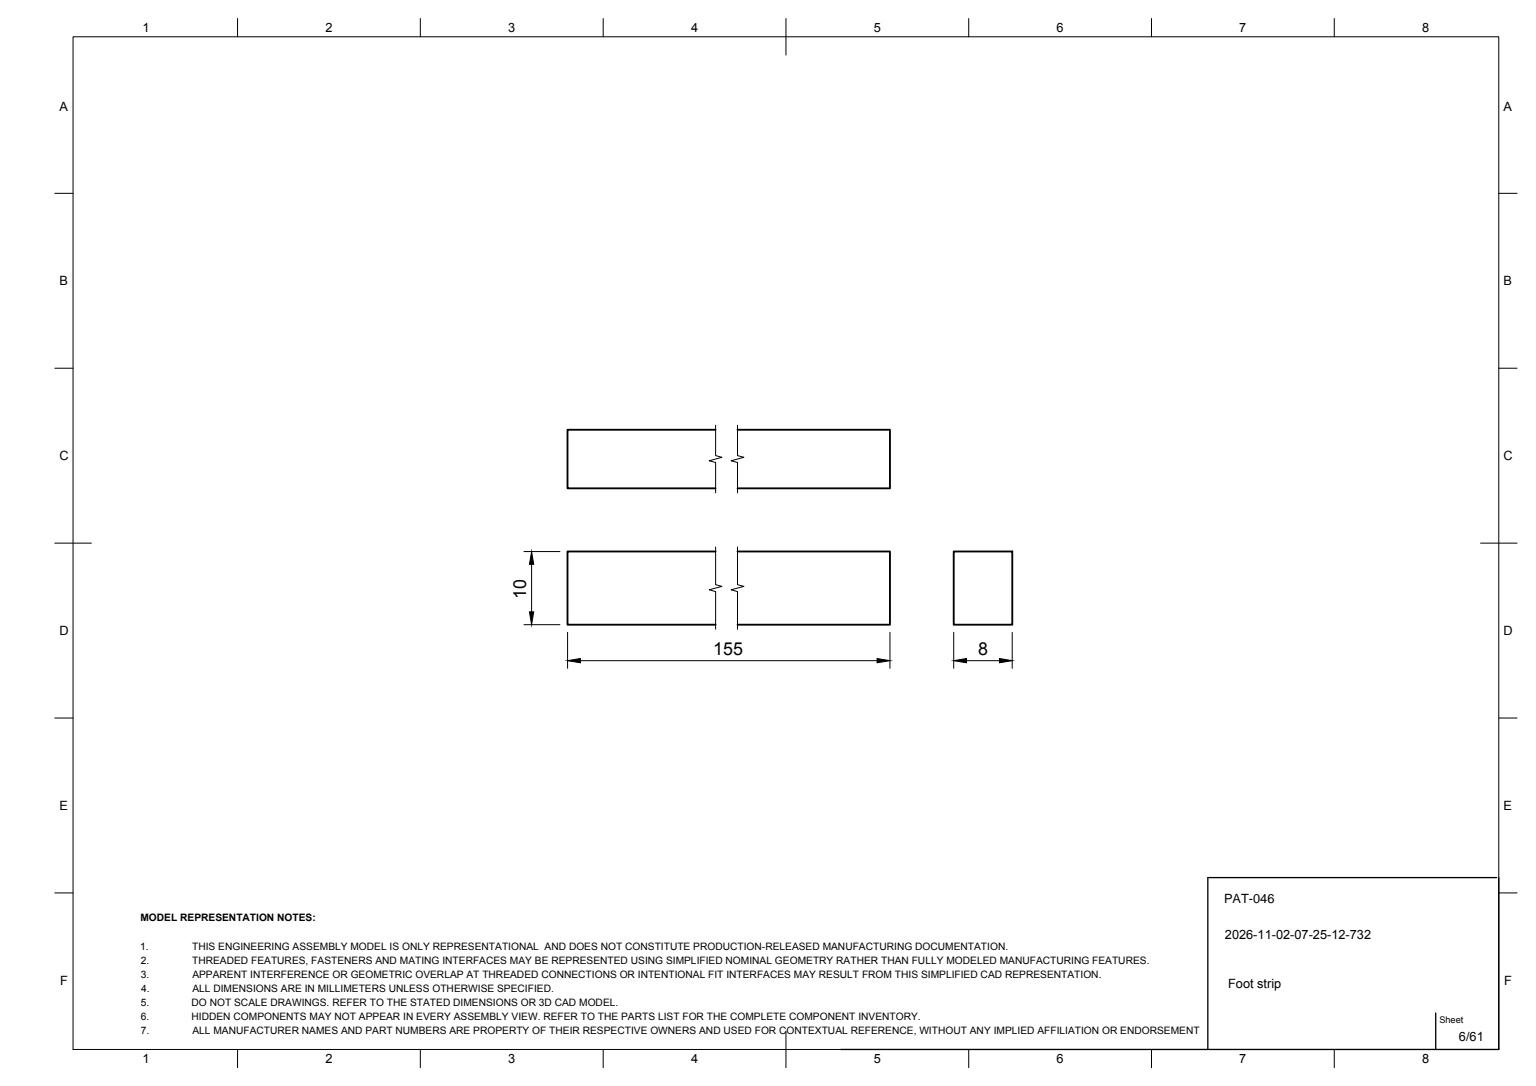
ISO-10303-21;
HEADER;
/* Generated by software containing ST-Developer
 * from STEP Tools, Inc. (www.steptools.com) 
 */

FILE_DESCRIPTION(
/* description */ ('Gear mesh backlash fixture'),
/* implementation_level */ '2;1');

FILE_NAME(
/* name */ 'Foot strip.step',
/* time_stamp */ '2026-10-28T03:26:00-07:00',
/* author */ (''),
/* organization */ (''),
/* preprocessor_version */ 'ST-DEVELOPER v20.2',
/* originating_system */ 'Autodesk Translation Framework v15.17.0.0',
/* authorisation */ '');

FILE_SCHEMA (('AUTOMOTIVE_DESIGN { 1 0 10303 214 3 1 1 }'));
ENDSEC;

DATA;
#10=MECHANICAL_DESIGN_GEOMETRIC_PRESENTATION_REPRESENTATION('',(#1017),#57900);
#917=SHAPE_REPRESENTATION_RELATIONSHIP('SRR','None',#58112,#967);
#967=ADVANCED_BREP_SHAPE_REPRESENTATION('',(#1082),#57845);
#1017=STYLED_ITEM('',(#58451),#1082);
#1082=MANIFOLD_SOLID_BREP('Body1',#13577);
#1336=PLANE('',#14241);
#1337=PLANE('',#14242);
#1338=PLANE('',#14243);
#1339=PLANE('',#14244);
#1340=PLANE('',#14245);
#1341=PLANE('',#14246);
#1712=FACE_OUTER_BOUND('',#2501,.T.);
#1713=FACE_OUTER_BOUND('',#2502,.T.);
#1714=FACE_OUTER_BOUND('',#2503,.T.);
#1715=FACE_OUTER_BOUND('',#2504,.T.);
#1716=FACE_OUTER_BOUND('',#2505,.T.);
#1717=FACE_OUTER_BOUND('',#2506,.T.);
#2501=EDGE_LOOP('',(#8975,#8976,#8977,#8978));
#2502=EDGE_LOOP('',(#8979,#8980,#8981,#8982));
#2503=EDGE_LOOP('',(#8983,#8984,#8985,#8986));
#2504=EDGE_LOOP('',(#8987,#8988,#8989,#8990));
#2505=EDGE_LOOP('',(#8991,#8992,#8993,#8994));
#2506=EDGE_LOOP('',(#8995,#8996,#8997,#8998));
#3435=LINE('',#19338,#4324);
#3436=LINE('',#19340,#4325);
#3437=LINE('',#19342,#4326);
#3438=LINE('',#19343,#4327);
#3439=LINE('',#19346,#4328);
#3440=LINE('',#19348,#4329);
#3441=LINE('',#19349,#4330);
#3442=LINE('',#19352,#4331);
#3443=LINE('',#19354,#4332);
#3444=LINE('',#19355,#4333);
#3445=LINE('',#19357,#4334);
#3446=LINE('',#19358,#4335);
#4324=VECTOR('',#15696,1.);
#4325=VECTOR('',#15697,1.);
#4326=VECTOR('',#15698,1.);
#4327=VECTOR('',#15699,1.);
#4328=VECTOR('',#15702,1.);
#4329=VECTOR('',#15703,1.);
#4330=VECTOR('',#15704,1.);
#4331=VECTOR('',#15707,1.);
#4332=VECTOR('',#15708,1.);
#4333=VECTOR('',#15709,1.);
#4334=VECTOR('',#15712,1.);
#4335=VECTOR('',#15713,1.);
#5813=VERTEX_POINT('',#19336);
#5814=VERTEX_POINT('',#19337);
#5815=VERTEX_POINT('',#19339);
#5816=VERTEX_POINT('',#19341);
#5817=VERTEX_POINT('',#19345);
#5818=VERTEX_POINT('',#19347);
#5819=VERTEX_POINT('',#19351);
#5820=VERTEX_POINT('',#19353);
#7074=EDGE_CURVE('',#5813,#5814,#3435,.T.);
#7075=EDGE_CURVE('',#5814,#5815,#3436,.T.);
#7076=EDGE_CURVE('',#5816,#5815,#3437,.T.);
#7077=EDGE_CURVE('',#5813,#5816,#3438,.T.);
#7078=EDGE_CURVE('',#5817,#5813,#3439,.T.);
#7079=EDGE_CURVE('',#5818,#5816,#3440,.T.);
#7080=EDGE_CURVE('',#5817,#5818,#3441,.T.);
#7081=EDGE_CURVE('',#5819,#5817,#3442,.T.);
#7082=EDGE_CURVE('',#5820,#5818,#3443,.T.);
#7083=EDGE_CURVE('',#5819,#5820,#3444,.T.);
#7084=EDGE_CURVE('',#5814,#5819,#3445,.T.);
#7085=EDGE_CURVE('',#5815,#5820,#3446,.T.);
#8975=ORIENTED_EDGE('',*,*,#7074,.T.);
#8976=ORIENTED_EDGE('',*,*,#7075,.T.);
#8977=ORIENTED_EDGE('',*,*,#7076,.F.);
#8978=ORIENTED_EDGE('',*,*,#7077,.F.);
#8979=ORIENTED_EDGE('',*,*,#7078,.T.);
#8980=ORIENTED_EDGE('',*,*,#7077,.T.);
#8981=ORIENTED_EDGE('',*,*,#7079,.F.);
#8982=ORIENTED_EDGE('',*,*,#7080,.F.);
#8983=ORIENTED_EDGE('',*,*,#7081,.T.);
#8984=ORIENTED_EDGE('',*,*,#7080,.T.);
#8985=ORIENTED_EDGE('',*,*,#7082,.F.);
#8986=ORIENTED_EDGE('',*,*,#7083,.F.);
#8987=ORIENTED_EDGE('',*,*,#7084,.T.);
#8988=ORIENTED_EDGE('',*,*,#7083,.T.);
#8989=ORIENTED_EDGE('',*,*,#7085,.F.);
#8990=ORIENTED_EDGE('',*,*,#7075,.F.);
#8991=ORIENTED_EDGE('',*,*,#7085,.T.);
#8992=ORIENTED_EDGE('',*,*,#7082,.T.);
#8993=ORIENTED_EDGE('',*,*,#7079,.T.);
#8994=ORIENTED_EDGE('',*,*,#7076,.T.);
#8995=ORIENTED_EDGE('',*,*,#7084,.F.);
#8996=ORIENTED_EDGE('',*,*,#7074,.F.);
#8997=ORIENTED_EDGE('',*,*,#7078,.F.);
#8998=ORIENTED_EDGE('',*,*,#7081,.F.);
#12829=ADVANCED_FACE('',(#1712),#1336,.T.);
#12830=ADVANCED_FACE('',(#1713),#1337,.T.);
#12831=ADVANCED_FACE('',(#1714),#1338,.T.);
#12832=ADVANCED_FACE('',(#1715),#1339,.T.);
#12833=ADVANCED_FACE('',(#1716),#1340,.T.);
#12834=ADVANCED_FACE('',(#1717),#1341,.F.);
#13577=CLOSED_SHELL('',(#12829,#12830,#12831,#12832,#12833,#12834));
#14240=AXIS2_PLACEMENT_3D('',#19334,#15692,#15693);
#14241=AXIS2_PLACEMENT_3D('',#19335,#15694,#15695);
#14242=AXIS2_PLACEMENT_3D('',#19344,#15700,#15701);
#14243=AXIS2_PLACEMENT_3D('',#19350,#15705,#15706);
#14244=AXIS2_PLACEMENT_3D('',#19356,#15710,#15711);
#14245=AXIS2_PLACEMENT_3D('',#19359,#15714,#15715);
#14246=AXIS2_PLACEMENT_3D('',#19360,#15716,#15717);
#15692=DIRECTION('axis',(0.,0.,1.));
#15693=DIRECTION('refdir',(1.,0.,0.));
#15694=DIRECTION('center_axis',(0.,1.,0.));
#15695=DIRECTION('ref_axis',(-1.,0.,0.));
#15696=DIRECTION('',(-1.,0.,0.));
#15697=DIRECTION('',(0.,0.,1.));
#15698=DIRECTION('',(-1.,0.,0.));
#15699=DIRECTION('',(0.,0.,1.));
#15700=DIRECTION('center_axis',(1.,0.,0.));
#15701=DIRECTION('ref_axis',(0.,1.,0.));
#15702=DIRECTION('',(0.,1.,0.));
#15703=DIRECTION('',(0.,1.,0.));
#15704=DIRECTION('',(0.,0.,1.));
#15705=DIRECTION('center_axis',(0.,-1.,0.));
#15706=DIRECTION('ref_axis',(1.,0.,0.));
#15707=DIRECTION('',(1.,0.,0.));
#15708=DIRECTION('',(1.,0.,0.));
#15709=DIRECTION('',(0.,0.,1.));
#15710=DIRECTION('center_axis',(-1.,0.,0.));
#15711=DIRECTION('ref_axis',(0.,-1.,0.));
#15712=DIRECTION('',(0.,-1.,0.));
#15713=DIRECTION('',(0.,-1.,0.));
#15714=DIRECTION('center_axis',(0.,0.,1.));
#15715=DIRECTION('ref_axis',(1.,0.,0.));
#15716=DIRECTION('center_axis',(0.,0.,1.));
#15717=DIRECTION('ref_axis',(1.,0.,0.));
#19334=CARTESIAN_POINT('',(0.,0.,0.));
#19335=CARTESIAN_POINT('Origin',(-2.5,11.5,-1.8));
#19336=CARTESIAN_POINT('',(-2.5,11.5,-1.8));
#19337=CARTESIAN_POINT('',(-3.5,11.5,-1.8));
#19338=CARTESIAN_POINT('',(-2.5,11.5,-1.8));
#19339=CARTESIAN_POINT('',(-3.5,11.5,-1.));
#19340=CARTESIAN_POINT('',(-3.5,11.5,-1.8));
#19341=CARTESIAN_POINT('',(-2.5,11.5,-1.));
#19342=CARTESIAN_POINT('',(-2.5,11.5,-1.));
#19343=CARTESIAN_POINT('',(-2.5,11.5,-1.8));
#19344=CARTESIAN_POINT('Origin',(-2.5,-4.,-1.8));
#19345=CARTESIAN_POINT('',(-2.5,-4.,-1.8));
#19346=CARTESIAN_POINT('',(-2.5,-4.,-1.8));
#19347=CARTESIAN_POINT('',(-2.5,-4.,-1.));
#19348=CARTESIAN_POINT('',(-2.5,-4.,-1.));
#19349=CARTESIAN_POINT('',(-2.5,-4.,-1.8));
#19350=CARTESIAN_POINT('Origin',(-3.5,-4.,-1.8));
#19351=CARTESIAN_POINT('',(-3.5,-4.,-1.8));
#19352=CARTESIAN_POINT('',(-3.5,-4.,-1.8));
#19353=CARTESIAN_POINT('',(-3.5,-4.,-1.));
#19354=CARTESIAN_POINT('',(-3.5,-4.,-1.));
#19355=CARTESIAN_POINT('',(-3.5,-4.,-1.8));
#19356=CARTESIAN_POINT('Origin',(-3.5,11.5,-1.8));
#19357=CARTESIAN_POINT('',(-3.5,11.5,-1.8));
#19358=CARTESIAN_POINT('',(-3.5,11.5,-1.));
#19359=CARTESIAN_POINT('Origin',(-3.,3.75,-1.));
#19360=CARTESIAN_POINT('Origin',(-3.,3.75,-1.8));
#57786=UNCERTAINTY_MEASURE_WITH_UNIT(LENGTH_MEASURE(0.001),#57901,
'DISTANCE_ACCURACY_VALUE',
'Maximum model space distance between geometric entities at asserted c
onnectivities');
#57841=UNCERTAINTY_MEASURE_WITH_UNIT(LENGTH_MEASURE(0.001),#57901,
'DISTANCE_ACCURACY_VALUE',
'Maximum model space distance between geometric entities at asserted c
onnectivities');
#57845=(
GEOMETRIC_REPRESENTATION_CONTEXT(3)
GLOBAL_UNCERTAINTY_ASSIGNED_CONTEXT((#57786))
GLOBAL_UNIT_ASSIGNED_CONTEXT((#57901,#57903,#57904))
REPRESENTATION_CONTEXT('','3D')
);
#57900=(
GEOMETRIC_REPRESENTATION_CONTEXT(3)
GLOBAL_UNCERTAINTY_ASSIGNED_CONTEXT((#57841))
GLOBAL_UNIT_ASSIGNED_CONTEXT((#57901,#57903,#57904))
REPRESENTATION_CONTEXT('','3D')
);
#57901=(
LENGTH_UNIT()
NAMED_UNIT(*)
SI_UNIT(.CENTI.,.METRE.)
);
#57903=(
NAMED_UNIT(*)
PLANE_ANGLE_UNIT()
SI_UNIT($,.RADIAN.)
);
#57904=(
NAMED_UNIT(*)
SI_UNIT($,.STERADIAN.)
SOLID_ANGLE_UNIT()
);
#57908=SHAPE_DEFINITION_REPRESENTATION(#57966,#58112);
#57966=PRODUCT_DEFINITION_SHAPE('',$,#58171);
#58112=SHAPE_REPRESENTATION('',(#14240),#57845);
#58167=PRODUCT_DEFINITION_CONTEXT('part definition',#58343,'design');
#58171=PRODUCT_DEFINITION('Foot strip','Foot strip',#58229,#58167);
#58229=PRODUCT_DEFINITION_FORMATION('',$,#58348);
#58343=APPLICATION_CONTEXT(
'Core Data for Automotive Mechanical Design Process');
#58344=PRODUCT_CONTEXT('part definition',#58343,'mechanical');
#58348=PRODUCT('Foot strip','Foot strip','Foot strip',(#58344));
#58445=COLOUR_RGB('Light Blue',0.38,0.62,0.78);
#58446=FILL_AREA_STYLE_COLOUR('',#58445);
#58447=FILL_AREA_STYLE('',(#58446));
#58448=SURFACE_STYLE_FILL_AREA(#58447);
#58449=SURFACE_SIDE_STYLE('',(#58448));
#58450=SURFACE_STYLE_USAGE(.BOTH.,#58449);
#58451=PRESENTATION_STYLE_ASSIGNMENT((#58450));
ENDSEC;
END-ISO-10303-21;
